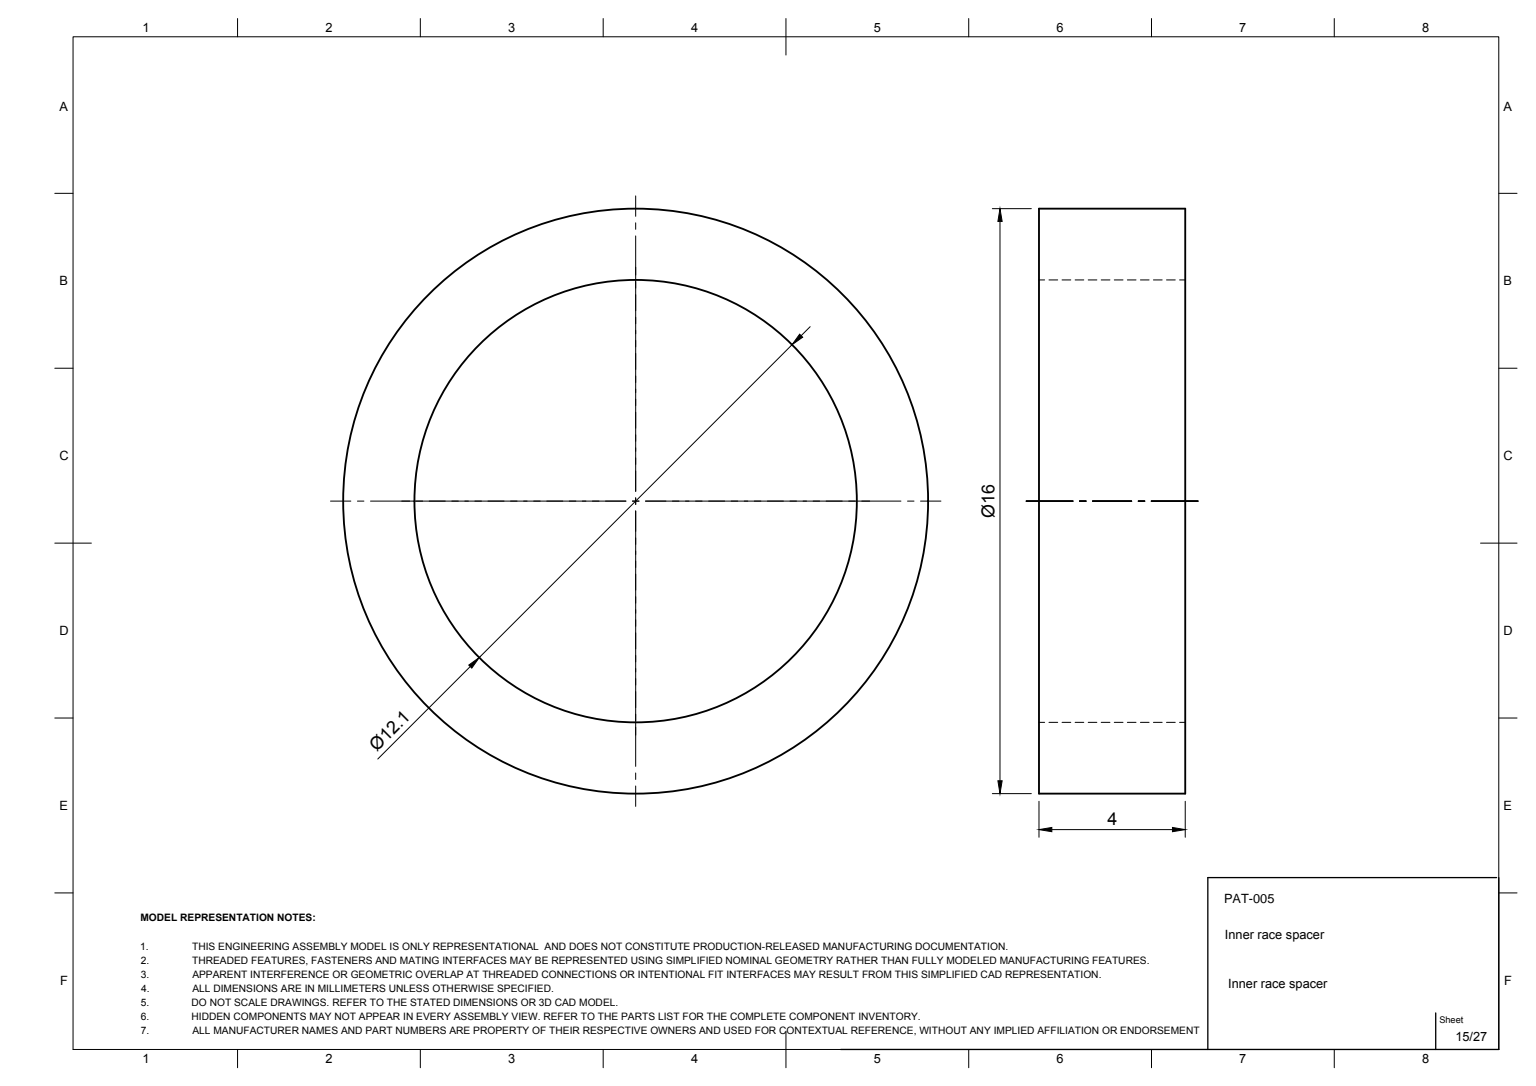
ISO-10303-21;
HEADER;
/* Generated by software containing ST-Developer
 * from STEP Tools, Inc. (www.steptools.com) 
 */

FILE_DESCRIPTION(
/* description */ ('Ball-race swivel caster'),
/* implementation_level */ '2;1');

FILE_NAME(
/* name */ 'Inner race spacer.step',
/* time_stamp */ '2026-10-29T16:15:51-07:00',
/* author */ (''),
/* organization */ (''),
/* preprocessor_version */ 'ST-DEVELOPER v20.2',
/* originating_system */ 'Autodesk Translation Framework v15.17.0.0',
/* authorisation */ '');

FILE_SCHEMA (('AUTOMOTIVE_DESIGN { 1 0 10303 214 3 1 1 }'));
ENDSEC;

DATA;
#10=MECHANICAL_DESIGN_GEOMETRIC_PRESENTATION_REPRESENTATION('',(#317),#7816);
#268=SHAPE_REPRESENTATION_RELATIONSHIP('SRR','None',#7915,#288);
#288=ADVANCED_BREP_SHAPE_REPRESENTATION('',(#353),#7804);
#317=STYLED_ITEM('',(#8097),#353);
#353=MANIFOLD_SOLID_BREP('Body1',#3723);
#418=FACE_BOUND('',#910,.T.);
#419=FACE_BOUND('',#912,.T.);
#487=PLANE('',#4284);
#488=PLANE('',#4285);
#649=FACE_OUTER_BOUND('',#907,.T.);
#650=FACE_OUTER_BOUND('',#908,.T.);
#651=FACE_OUTER_BOUND('',#909,.T.);
#652=FACE_OUTER_BOUND('',#911,.T.);
#907=EDGE_LOOP('',(#3109,#3110,#3111,#3112));
#908=EDGE_LOOP('',(#3113,#3114,#3115,#3116));
#909=EDGE_LOOP('',(#3117));
#910=EDGE_LOOP('',(#3118));
#911=EDGE_LOOP('',(#3119));
#912=EDGE_LOOP('',(#3120));
#1117=LINE('',#7086,#1272);
#1118=LINE('',#7092,#1273);
#1272=VECTOR('',#5231,0.605);
#1273=VECTOR('',#5238,0.8);
#1489=CIRCLE('',#4279,0.605);
#1490=CIRCLE('',#4280,0.605);
#1491=CIRCLE('',#4282,0.8);
#1492=CIRCLE('',#4283,0.8);
#1823=VERTEX_POINT('',#7083);
#1824=VERTEX_POINT('',#7085);
#1825=VERTEX_POINT('',#7089);
#1826=VERTEX_POINT('',#7091);
#2274=EDGE_CURVE('',#1823,#1823,#1489,.T.);
#2275=EDGE_CURVE('',#1823,#1824,#1117,.T.);
#2276=EDGE_CURVE('',#1824,#1824,#1490,.T.);
#2277=EDGE_CURVE('',#1825,#1825,#1491,.T.);
#2278=EDGE_CURVE('',#1825,#1826,#1118,.T.);
#2279=EDGE_CURVE('',#1826,#1826,#1492,.T.);
#3109=ORIENTED_EDGE('',*,*,#2274,.F.);
#3110=ORIENTED_EDGE('',*,*,#2275,.T.);
#3111=ORIENTED_EDGE('',*,*,#2276,.T.);
#3112=ORIENTED_EDGE('',*,*,#2275,.F.);
#3113=ORIENTED_EDGE('',*,*,#2277,.F.);
#3114=ORIENTED_EDGE('',*,*,#2278,.T.);
#3115=ORIENTED_EDGE('',*,*,#2279,.T.);
#3116=ORIENTED_EDGE('',*,*,#2278,.F.);
#3117=ORIENTED_EDGE('',*,*,#2277,.T.);
#3118=ORIENTED_EDGE('',*,*,#2274,.T.);
#3119=ORIENTED_EDGE('',*,*,#2279,.F.);
#3120=ORIENTED_EDGE('',*,*,#2276,.F.);
#3471=CYLINDRICAL_SURFACE('',#4278,0.605);
#3472=CYLINDRICAL_SURFACE('',#4281,0.8);
#3620=ADVANCED_FACE('',(#649),#3471,.F.);
#3621=ADVANCED_FACE('',(#650),#3472,.T.);
#3622=ADVANCED_FACE('',(#651,#418),#487,.T.);
#3623=ADVANCED_FACE('',(#652,#419),#488,.F.);
#3723=CLOSED_SHELL('',(#3620,#3621,#3622,#3623));
#4277=AXIS2_PLACEMENT_3D('',#7081,#5225,#5226);
#4278=AXIS2_PLACEMENT_3D('',#7082,#5227,#5228);
#4279=AXIS2_PLACEMENT_3D('',#7084,#5229,#5230);
#4280=AXIS2_PLACEMENT_3D('',#7087,#5232,#5233);
#4281=AXIS2_PLACEMENT_3D('',#7088,#5234,#5235);
#4282=AXIS2_PLACEMENT_3D('',#7090,#5236,#5237);
#4283=AXIS2_PLACEMENT_3D('',#7093,#5239,#5240);
#4284=AXIS2_PLACEMENT_3D('',#7094,#5241,#5242);
#4285=AXIS2_PLACEMENT_3D('',#7095,#5243,#5244);
#5225=DIRECTION('axis',(0.,0.,1.));
#5226=DIRECTION('refdir',(1.,0.,0.));
#5227=DIRECTION('center_axis',(0.,1.,0.));
#5228=DIRECTION('ref_axis',(1.,0.,0.));
#5229=DIRECTION('center_axis',(0.,-1.,0.));
#5230=DIRECTION('ref_axis',(1.,0.,0.));
#5231=DIRECTION('',(0.,-1.,0.));
#5232=DIRECTION('center_axis',(0.,-1.,0.));
#5233=DIRECTION('ref_axis',(1.,0.,0.));
#5234=DIRECTION('center_axis',(0.,1.,0.));
#5235=DIRECTION('ref_axis',(1.,0.,0.));
#5236=DIRECTION('center_axis',(0.,1.,0.));
#5237=DIRECTION('ref_axis',(1.,0.,0.));
#5238=DIRECTION('',(0.,-1.,0.));
#5239=DIRECTION('center_axis',(0.,1.,0.));
#5240=DIRECTION('ref_axis',(1.,0.,0.));
#5241=DIRECTION('center_axis',(0.,1.,0.));
#5242=DIRECTION('ref_axis',(1.,0.,0.));
#5243=DIRECTION('center_axis',(0.,1.,0.));
#5244=DIRECTION('ref_axis',(1.,0.,0.));
#7081=CARTESIAN_POINT('',(0.,0.,0.));
#7082=CARTESIAN_POINT('Origin',(0.,4.5,10.));
#7083=CARTESIAN_POINT('',(-0.605,4.9,10.));
#7084=CARTESIAN_POINT('Origin',(0.,4.9,10.));
#7085=CARTESIAN_POINT('',(-0.605,4.5,10.));
#7086=CARTESIAN_POINT('',(-0.605,4.5,10.));
#7087=CARTESIAN_POINT('Origin',(0.,4.5,10.));
#7088=CARTESIAN_POINT('Origin',(0.,4.5,10.));
#7089=CARTESIAN_POINT('',(-0.8,4.9,10.));
#7090=CARTESIAN_POINT('Origin',(0.,4.9,10.));
#7091=CARTESIAN_POINT('',(-0.8,4.5,10.));
#7092=CARTESIAN_POINT('',(-0.8,4.5,10.));
#7093=CARTESIAN_POINT('Origin',(0.,4.5,10.));
#7094=CARTESIAN_POINT('Origin',(0.,4.9,10.));
#7095=CARTESIAN_POINT('Origin',(0.,4.5,10.));
#7777=UNCERTAINTY_MEASURE_WITH_UNIT(LENGTH_MEASURE(0.001),#7817,
'DISTANCE_ACCURACY_VALUE',
'Maximum model space distance between geometric entities at asserted c
onnectivities');
#7789=UNCERTAINTY_MEASURE_WITH_UNIT(LENGTH_MEASURE(0.001),#7817,
'DISTANCE_ACCURACY_VALUE',
'Maximum model space distance between geometric entities at asserted c
onnectivities');
#7804=(
GEOMETRIC_REPRESENTATION_CONTEXT(3)
GLOBAL_UNCERTAINTY_ASSIGNED_CONTEXT((#7777))
GLOBAL_UNIT_ASSIGNED_CONTEXT((#7817,#7819,#7820))
REPRESENTATION_CONTEXT('','3D')
);
#7816=(
GEOMETRIC_REPRESENTATION_CONTEXT(3)
GLOBAL_UNCERTAINTY_ASSIGNED_CONTEXT((#7789))
GLOBAL_UNIT_ASSIGNED_CONTEXT((#7817,#7819,#7820))
REPRESENTATION_CONTEXT('','3D')
);
#7817=(
LENGTH_UNIT()
NAMED_UNIT(*)
SI_UNIT(.CENTI.,.METRE.)
);
#7819=(
NAMED_UNIT(*)
PLANE_ANGLE_UNIT()
SI_UNIT($,.RADIAN.)
);
#7820=(
NAMED_UNIT(*)
SI_UNIT($,.STERADIAN.)
SOLID_ANGLE_UNIT()
);
#7835=SHAPE_DEFINITION_REPRESENTATION(#7869,#7915);
#7869=PRODUCT_DEFINITION_SHAPE('',$,#7942);
#7915=SHAPE_REPRESENTATION('',(#4277),#7804);
#7927=PRODUCT_DEFINITION_CONTEXT('part definition',#8007,'design');
#7942=PRODUCT_DEFINITION('Inner race spacer','Inner race spacer',#7968,
#7927);
#7968=PRODUCT_DEFINITION_FORMATION('',$,#8023);
#8007=APPLICATION_CONTEXT(
'Core Data for Automotive Mechanical Design Process');
#8008=PRODUCT_CONTEXT('part definition',#8007,'mechanical');
#8023=PRODUCT('Inner race spacer','Inner race spacer',
'Inner race spacer',(#8008));
#8091=COLOUR_RGB('Grey',0.48,0.52,0.57);
#8092=FILL_AREA_STYLE_COLOUR('',#8091);
#8093=FILL_AREA_STYLE('',(#8092));
#8094=SURFACE_STYLE_FILL_AREA(#8093);
#8095=SURFACE_SIDE_STYLE('',(#8094));
#8096=SURFACE_STYLE_USAGE(.BOTH.,#8095);
#8097=PRESENTATION_STYLE_ASSIGNMENT((#8096));
ENDSEC;
END-ISO-10303-21;
